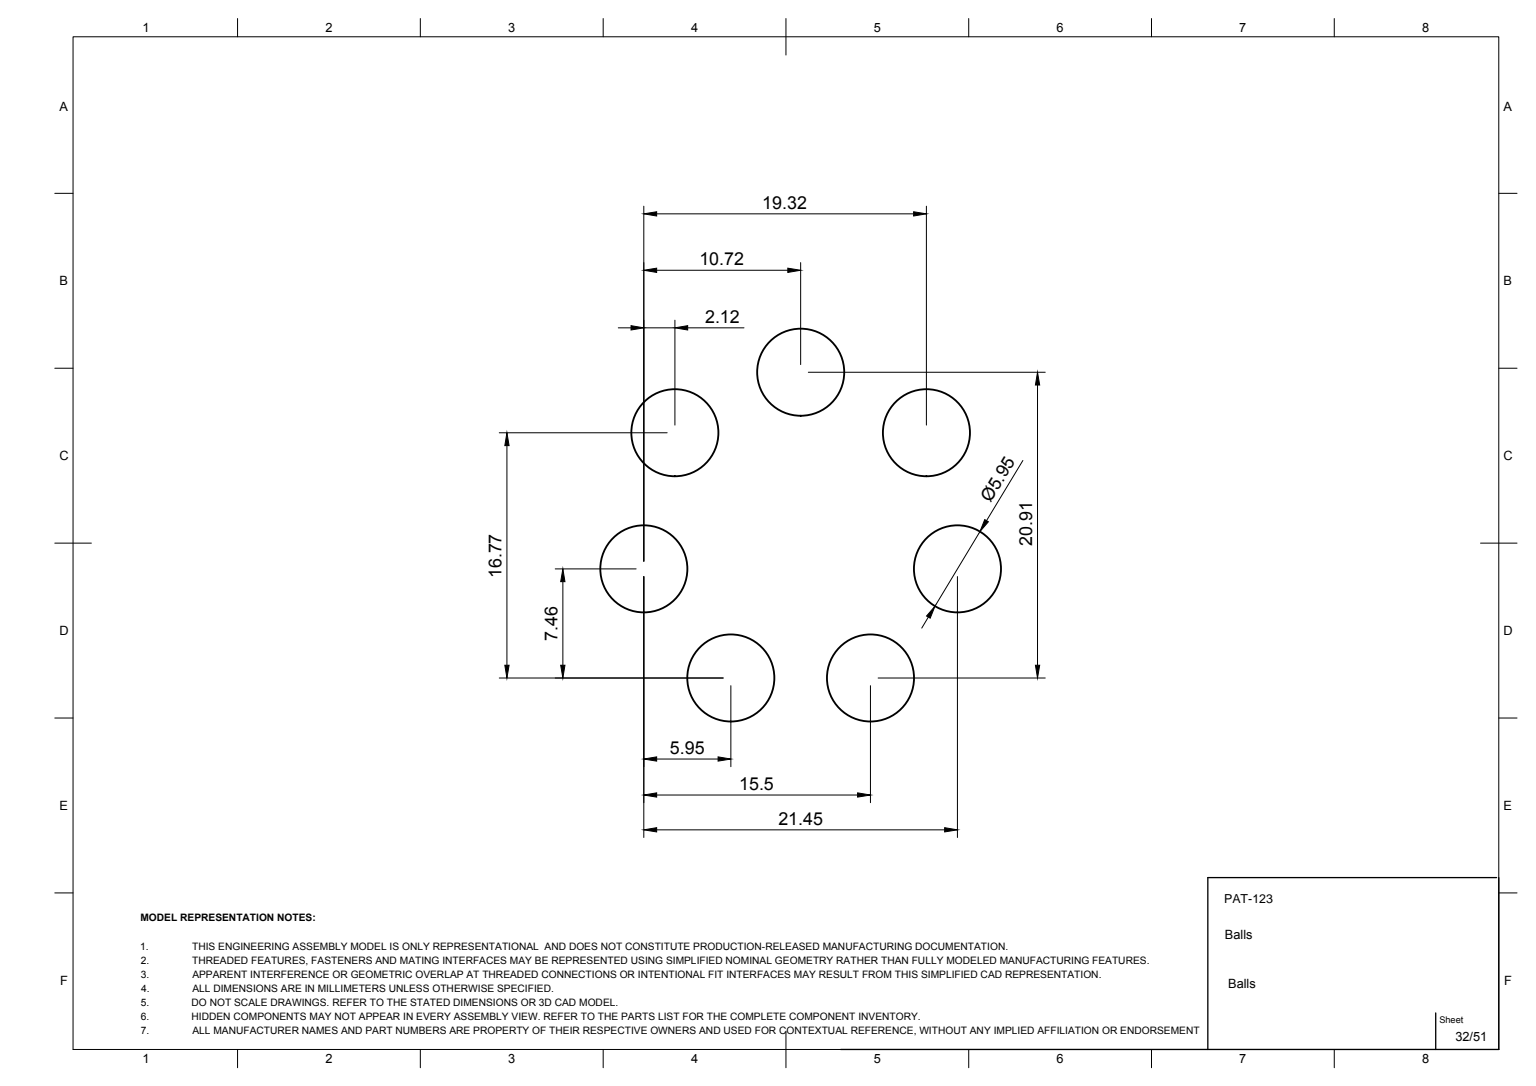
ISO-10303-21;
HEADER;
/* Generated by software containing ST-Developer
 * from STEP Tools, Inc. (www.steptools.com) 
 */

FILE_DESCRIPTION(
/* description */ ('Worm-less right-angle friction wheel drive'),
/* implementation_level */ '2;1');

FILE_NAME(
/* name */ 'Balls.step',
/* time_stamp */ '2026-10-28T03:22:36-07:00',
/* author */ (''),
/* organization */ (''),
/* preprocessor_version */ 'ST-DEVELOPER v20.2',
/* originating_system */ 'Autodesk Translation Framework v15.17.0.0',
/* authorisation */ '');

FILE_SCHEMA (('AUTOMOTIVE_DESIGN { 1 0 10303 214 3 1 1 }'));
ENDSEC;

DATA;
#10=MECHANICAL_DESIGN_GEOMETRIC_PRESENTATION_REPRESENTATION('',(#637,#638,#639,#640,#641,#642,#643),#17046);
#435=SPHERICAL_SURFACE('',#9303,0.29765);
#436=SPHERICAL_SURFACE('',#9305,0.29765);
#437=SPHERICAL_SURFACE('',#9307,0.29765);
#438=SPHERICAL_SURFACE('',#9309,0.29765);
#439=SPHERICAL_SURFACE('',#9311,0.29765);
#440=SPHERICAL_SURFACE('',#9313,0.29765);
#441=SPHERICAL_SURFACE('',#9315,0.29765);
#543=SHAPE_REPRESENTATION_RELATIONSHIP('SRR','None',#17287,#590);
#590=ADVANCED_BREP_SHAPE_REPRESENTATION('',(#690,#691,#692,#693,#694,#695,
#696),#17023);
#637=STYLED_ITEM('',(#17591),#690);
#638=STYLED_ITEM('',(#17591),#691);
#639=STYLED_ITEM('',(#17591),#692);
#640=STYLED_ITEM('',(#17591),#693);
#641=STYLED_ITEM('',(#17591),#694);
#642=STYLED_ITEM('',(#17591),#695);
#643=STYLED_ITEM('',(#17591),#696);
#690=MANIFOLD_SOLID_BREP('Body1',#8193);
#691=MANIFOLD_SOLID_BREP('Body2',#8194);
#692=MANIFOLD_SOLID_BREP('Body3',#8195);
#693=MANIFOLD_SOLID_BREP('Body4',#8196);
#694=MANIFOLD_SOLID_BREP('Body5',#8197);
#695=MANIFOLD_SOLID_BREP('Body6',#8198);
#696=MANIFOLD_SOLID_BREP('Body7',#8199);
#1475=FACE_OUTER_BOUND('',#2136,.T.);
#1476=FACE_OUTER_BOUND('',#2137,.T.);
#1477=FACE_OUTER_BOUND('',#2138,.T.);
#1478=FACE_OUTER_BOUND('',#2139,.T.);
#1479=FACE_OUTER_BOUND('',#2140,.T.);
#1480=FACE_OUTER_BOUND('',#2141,.T.);
#1481=FACE_OUTER_BOUND('',#2142,.T.);
#2136=EDGE_LOOP('',(#6730,#6731));
#2137=EDGE_LOOP('',(#6732,#6733));
#2138=EDGE_LOOP('',(#6734,#6735));
#2139=EDGE_LOOP('',(#6736,#6737));
#2140=EDGE_LOOP('',(#6738,#6739));
#2141=EDGE_LOOP('',(#6740,#6741));
#2142=EDGE_LOOP('',(#6742,#6743));
#3723=CIRCLE('',#9304,0.29765);
#3724=CIRCLE('',#9306,0.29765);
#3725=CIRCLE('',#9308,0.29765);
#3726=CIRCLE('',#9310,0.29765);
#3727=CIRCLE('',#9312,0.29765);
#3728=CIRCLE('',#9314,0.29765);
#3729=CIRCLE('',#9316,0.29765);
#4265=VERTEX_POINT('',#15467);
#4266=VERTEX_POINT('',#15468);
#4267=VERTEX_POINT('',#15471);
#4268=VERTEX_POINT('',#15472);
#4269=VERTEX_POINT('',#15475);
#4270=VERTEX_POINT('',#15476);
#4271=VERTEX_POINT('',#15479);
#4272=VERTEX_POINT('',#15480);
#4273=VERTEX_POINT('',#15483);
#4274=VERTEX_POINT('',#15484);
#4275=VERTEX_POINT('',#15487);
#4276=VERTEX_POINT('',#15488);
#4277=VERTEX_POINT('',#15491);
#4278=VERTEX_POINT('',#15492);
#5134=EDGE_CURVE('',#4265,#4266,#3723,.T.);
#5135=EDGE_CURVE('',#4267,#4268,#3724,.T.);
#5136=EDGE_CURVE('',#4269,#4270,#3725,.T.);
#5137=EDGE_CURVE('',#4271,#4272,#3726,.T.);
#5138=EDGE_CURVE('',#4273,#4274,#3727,.T.);
#5139=EDGE_CURVE('',#4275,#4276,#3728,.T.);
#5140=EDGE_CURVE('',#4277,#4278,#3729,.T.);
#6730=ORIENTED_EDGE('',*,*,#5134,.T.);
#6731=ORIENTED_EDGE('',*,*,#5134,.F.);
#6732=ORIENTED_EDGE('',*,*,#5135,.T.);
#6733=ORIENTED_EDGE('',*,*,#5135,.F.);
#6734=ORIENTED_EDGE('',*,*,#5136,.T.);
#6735=ORIENTED_EDGE('',*,*,#5136,.F.);
#6736=ORIENTED_EDGE('',*,*,#5137,.T.);
#6737=ORIENTED_EDGE('',*,*,#5137,.F.);
#6738=ORIENTED_EDGE('',*,*,#5138,.T.);
#6739=ORIENTED_EDGE('',*,*,#5138,.F.);
#6740=ORIENTED_EDGE('',*,*,#5139,.T.);
#6741=ORIENTED_EDGE('',*,*,#5139,.F.);
#6742=ORIENTED_EDGE('',*,*,#5140,.T.);
#6743=ORIENTED_EDGE('',*,*,#5140,.F.);
#7967=ADVANCED_FACE('',(#1475),#435,.T.);
#7968=ADVANCED_FACE('',(#1476),#436,.T.);
#7969=ADVANCED_FACE('',(#1477),#437,.T.);
#7970=ADVANCED_FACE('',(#1478),#438,.T.);
#7971=ADVANCED_FACE('',(#1479),#439,.T.);
#7972=ADVANCED_FACE('',(#1480),#440,.T.);
#7973=ADVANCED_FACE('',(#1481),#441,.T.);
#8193=CLOSED_SHELL('',(#7967));
#8194=CLOSED_SHELL('',(#7968));
#8195=CLOSED_SHELL('',(#7969));
#8196=CLOSED_SHELL('',(#7970));
#8197=CLOSED_SHELL('',(#7971));
#8198=CLOSED_SHELL('',(#7972));
#8199=CLOSED_SHELL('',(#7973));
#9302=AXIS2_PLACEMENT_3D('',#15465,#11223,#11224);
#9303=AXIS2_PLACEMENT_3D('',#15466,#11225,#11226);
#9304=AXIS2_PLACEMENT_3D('',#15469,#11227,#11228);
#9305=AXIS2_PLACEMENT_3D('',#15470,#11229,#11230);
#9306=AXIS2_PLACEMENT_3D('',#15473,#11231,#11232);
#9307=AXIS2_PLACEMENT_3D('',#15474,#11233,#11234);
#9308=AXIS2_PLACEMENT_3D('',#15477,#11235,#11236);
#9309=AXIS2_PLACEMENT_3D('',#15478,#11237,#11238);
#9310=AXIS2_PLACEMENT_3D('',#15481,#11239,#11240);
#9311=AXIS2_PLACEMENT_3D('',#15482,#11241,#11242);
#9312=AXIS2_PLACEMENT_3D('',#15485,#11243,#11244);
#9313=AXIS2_PLACEMENT_3D('',#15486,#11245,#11246);
#9314=AXIS2_PLACEMENT_3D('',#15489,#11247,#11248);
#9315=AXIS2_PLACEMENT_3D('',#15490,#11249,#11250);
#9316=AXIS2_PLACEMENT_3D('',#15493,#11251,#11252);
#11223=DIRECTION('axis',(0.,0.,1.));
#11224=DIRECTION('refdir',(1.,0.,0.));
#11225=DIRECTION('center_axis',(0.,0.,1.));
#11226=DIRECTION('ref_axis',(1.,0.,0.));
#11227=DIRECTION('center_axis',(1.22464679914735E-16,-1.,0.));
#11228=DIRECTION('ref_axis',(-1.,-1.22464679914735E-16,0.));
#11229=DIRECTION('center_axis',(0.78183148246803,0.,0.623489801858733));
#11230=DIRECTION('ref_axis',(0.623489801858734,0.,-0.78183148246803));
#11231=DIRECTION('center_axis',(7.63554790147315E-17,-1.,-9.57467422477103E-17));
#11232=DIRECTION('ref_axis',(-0.623489801858734,-1.22464679914735E-16,0.78183148246803));
#11233=DIRECTION('center_axis',(0.974927912181824,0.,-0.222520933956314));
#11234=DIRECTION('ref_axis',(-0.222520933956314,0.,-0.974927912181824));
#11235=DIRECTION('center_axis',(-2.7250954951288E-17,-1.,-1.19394234705288E-16));
#11236=DIRECTION('ref_axis',(0.222520933956314,-1.22464679914735E-16,0.974927912181824));
#11237=DIRECTION('center_axis',(0.433883739117558,0.,-0.900968867902419));
#11238=DIRECTION('ref_axis',(-0.900968867902419,0.,-0.433883739117558));
#11239=DIRECTION('center_axis',(-1.10336864020811E-16,-1.,-5.31354332312403E-17));
#11240=DIRECTION('ref_axis',(0.900968867902419,-1.22464679914735E-16,0.433883739117558));
#11241=DIRECTION('center_axis',(-0.433883739117558,0.,-0.900968867902419));
#11242=DIRECTION('ref_axis',(-0.900968867902419,0.,0.433883739117558));
#11243=DIRECTION('center_axis',(-1.10336864020811E-16,-1.,5.31354332312403E-17));
#11244=DIRECTION('ref_axis',(0.900968867902419,-1.22464679914735E-16,-0.433883739117558));
#11245=DIRECTION('center_axis',(-0.974927912181824,0.,-0.222520933956314));
#11246=DIRECTION('ref_axis',(-0.222520933956315,0.,0.974927912181824));
#11247=DIRECTION('center_axis',(-2.7250954951288E-17,-1.,1.19394234705288E-16));
#11248=DIRECTION('ref_axis',(0.222520933956315,-1.22464679914735E-16,-0.974927912181824));
#11249=DIRECTION('center_axis',(-0.78183148246803,0.,0.623489801858734));
#11250=DIRECTION('ref_axis',(0.623489801858733,0.,0.78183148246803));
#11251=DIRECTION('center_axis',(7.63554790147315E-17,-1.,9.57467422477103E-17));
#11252=DIRECTION('ref_axis',(-0.623489801858733,-1.22464679914735E-16,-0.78183148246803));
#15465=CARTESIAN_POINT('',(0.,0.,0.));
#15466=CARTESIAN_POINT('Origin',(1.1,0.,0.));
#15467=CARTESIAN_POINT('',(1.1,-2.23201749654651E-33,0.29765));
#15468=CARTESIAN_POINT('',(1.1,-2.23201749654651E-33,-0.29765));
#15469=CARTESIAN_POINT('Origin',(1.1,0.,0.));
#15470=CARTESIAN_POINT('Origin',(0.685838782044607,0.,-0.860014630714833));
#15471=CARTESIAN_POINT('',(0.918550922801216,-5.31350540756609E-33,-0.674432891191581));
#15472=CARTESIAN_POINT('',(0.453126641287998,8.49470414473068E-34,-1.04559637023808));
#15473=CARTESIAN_POINT('Origin',(0.685838782044607,0.,-0.860014630714833));
#15474=CARTESIAN_POINT('Origin',(-0.244773027351946,0.,-1.07242070340001));
#15475=CARTESIAN_POINT('',(0.0454142657089739,-2.23201749654651E-33,-1.1386540593921));
#15476=CARTESIAN_POINT('',(-0.534960320412865,-2.23201749654651E-33,-1.00618734740791));
#15477=CARTESIAN_POINT('Origin',(-0.244773027351946,0.,-1.07242070340001));
#15478=CARTESIAN_POINT('Origin',(-0.991065754692661,0.,-0.477272113029314));
#15479=CARTESIAN_POINT('',(-0.86192025974432,8.49470414473067E-34,-0.745445496560469));
#15480=CARTESIAN_POINT('',(-1.120211249641,-5.31350540756609E-33,-0.209098729498159));
#15481=CARTESIAN_POINT('Origin',(-0.991065754692661,0.,-0.477272113029314));
#15482=CARTESIAN_POINT('Origin',(-0.991065754692661,0.,0.477272113029314));
#15483=CARTESIAN_POINT('',(-1.120211249641,-2.23201749654651E-33,0.209098729498159));
#15484=CARTESIAN_POINT('',(-0.86192025974432,-2.23201749654651E-33,0.745445496560469));
#15485=CARTESIAN_POINT('Origin',(-0.991065754692661,0.,0.477272113029314));
#15486=CARTESIAN_POINT('Origin',(-0.244773027351946,0.,1.07242070340001));
#15487=CARTESIAN_POINT('',(-0.534960320412866,-2.23201749654651E-33,1.00618734740791));
#15488=CARTESIAN_POINT('',(0.0454142657089737,-2.23201749654651E-33,1.1386540593921));
#15489=CARTESIAN_POINT('Origin',(-0.244773027351946,0.,1.07242070340001));
#15490=CARTESIAN_POINT('Origin',(0.685838782044607,0.,0.860014630714833));
#15491=CARTESIAN_POINT('',(0.453126641287998,-2.23201749654651E-33,1.04559637023808));
#15492=CARTESIAN_POINT('',(0.918550922801216,-2.23201749654651E-33,0.674432891191581));
#15493=CARTESIAN_POINT('Origin',(0.685838782044607,0.,0.860014630714833));
#16970=UNCERTAINTY_MEASURE_WITH_UNIT(LENGTH_MEASURE(0.001),#17047,
'DISTANCE_ACCURACY_VALUE',
'Maximum model space distance between geometric entities at asserted c
onnectivities');
#16993=UNCERTAINTY_MEASURE_WITH_UNIT(LENGTH_MEASURE(0.001),#17047,
'DISTANCE_ACCURACY_VALUE',
'Maximum model space distance between geometric entities at asserted c
onnectivities');
#17023=(
GEOMETRIC_REPRESENTATION_CONTEXT(3)
GLOBAL_UNCERTAINTY_ASSIGNED_CONTEXT((#16970))
GLOBAL_UNIT_ASSIGNED_CONTEXT((#17047,#17049,#17050))
REPRESENTATION_CONTEXT('','3D')
);
#17046=(
GEOMETRIC_REPRESENTATION_CONTEXT(3)
GLOBAL_UNCERTAINTY_ASSIGNED_CONTEXT((#16993))
GLOBAL_UNIT_ASSIGNED_CONTEXT((#17047,#17049,#17050))
REPRESENTATION_CONTEXT('','3D')
);
#17047=(
LENGTH_UNIT()
NAMED_UNIT(*)
SI_UNIT(.CENTI.,.METRE.)
);
#17049=(
NAMED_UNIT(*)
PLANE_ANGLE_UNIT()
SI_UNIT($,.RADIAN.)
);
#17050=(
NAMED_UNIT(*)
SI_UNIT($,.STERADIAN.)
SOLID_ANGLE_UNIT()
);
#17080=SHAPE_DEFINITION_REPRESENTATION(#17132,#17287);
#17132=PRODUCT_DEFINITION_SHAPE('',$,#17340);
#17287=SHAPE_REPRESENTATION('',(#9302),#17023);
#17310=PRODUCT_DEFINITION_CONTEXT('part definition',#17468,'design');
#17340=PRODUCT_DEFINITION('Balls','Balls',#17392,#17310);
#17392=PRODUCT_DEFINITION_FORMATION('',$,#17499);
#17468=APPLICATION_CONTEXT(
'Core Data for Automotive Mechanical Design Process');
#17469=PRODUCT_CONTEXT('part definition',#17468,'mechanical');
#17499=PRODUCT('Balls','Balls','Balls',(#17469));
#17585=COLOUR_RGB('Grey',0.48,0.52,0.57);
#17586=FILL_AREA_STYLE_COLOUR('',#17585);
#17587=FILL_AREA_STYLE('',(#17586));
#17588=SURFACE_STYLE_FILL_AREA(#17587);
#17589=SURFACE_SIDE_STYLE('',(#17588));
#17590=SURFACE_STYLE_USAGE(.BOTH.,#17589);
#17591=PRESENTATION_STYLE_ASSIGNMENT((#17590));
ENDSEC;
END-ISO-10303-21;
